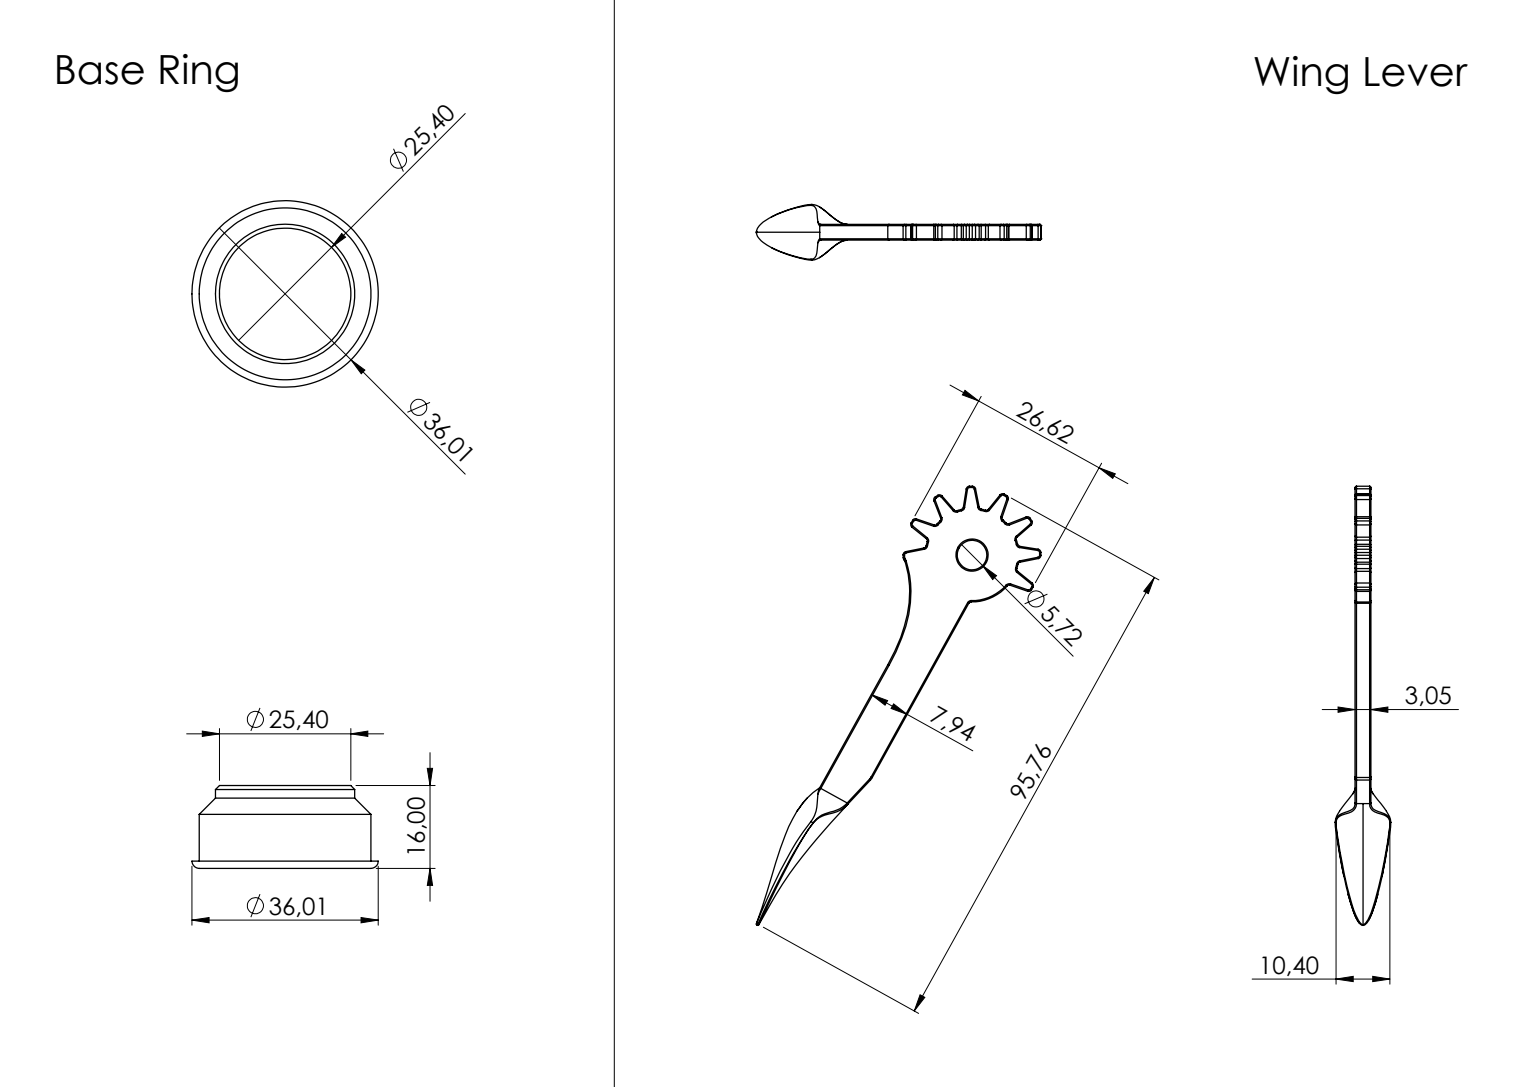
ISO-10303-21;
HEADER;
FILE_DESCRIPTION (('STEP AP214'),
    '1' );
FILE_NAME ('Base Ring.step',
    '2026-10-06T14:27:08',
    ( '' ),
    ( '' ),
    'SwSTEP 2.0',
    'SolidWorks 2020',
    '' );
FILE_SCHEMA (( 'AUTOMOTIVE_DESIGN' ));
ENDSEC;

DATA;
#28=SHAPE_DEFINITION_REPRESENTATION ( #10271, #23419 ) ;
#104=EDGE_LOOP ( 'NONE', ( #16225, #25822, #7892, #35896 ) ) ;
#162=DIRECTION ( 'NONE',  ( -1.000000000000000000, 1.365923996832131856E-16, 0.000000000000000000 ) ) ;
#198=EDGE_CURVE ( 'NONE', #31926, #33162, #2052, .T. ) ;
#286=EDGE_LOOP ( 'NONE', ( #24202, #14041, #34463, #28082 ) ) ;
#492=CONICAL_SURFACE ( 'NONE', #1854, 13.46199999999999619, 0.7853981633974482790 ) ;
#533=DIRECTION ( 'NONE',  ( -1.000000000000000000, 1.011795553208986377E-16, 0.000000000000000000 ) ) ;
#578=( GEOMETRIC_REPRESENTATION_CONTEXT ( 3 ) GLOBAL_UNCERTAINTY_ASSIGNED_CONTEXT ( ( #38497 ) ) GLOBAL_UNIT_ASSIGNED_CONTEXT ( ( #8767, #25159, #21514 ) ) REPRESENTATION_CONTEXT ( 'NONE', 'WORKASPACE' ) );
#588=VERTEX_POINT ( 'NONE', #40151 ) ;
#941=DIRECTION ( 'NONE',  ( -0.7071067811865480168, -0.7071067811865470176, 8.659560562354937789E-17 ) ) ;
#958=EDGE_LOOP ( 'NONE', ( #31328, #8348, #40597, #40431 ) ) ;
#1091=DIRECTION ( 'NONE',  ( 1.011795553208986377E-16, 1.000000000000000000, -0.000000000000000000 ) ) ;
#1122=FACE_OUTER_BOUND ( 'NONE', #9226, .T. ) ;
#1125=PRODUCT ( 'Base Ring', 'Base Ring', '', ( #16178 ) ) ;
#1185=CIRCLE ( 'NONE', #18138, 15.21260244842765452 ) ;
#1237=APPLICATION_CONTEXT ( 'automotive_design' ) ;
#1281=DIRECTION ( 'NONE',  ( 1.011795553208986377E-16, 1.000000000000000000, -0.000000000000000000 ) ) ;
#1340=CIRCLE ( 'NONE', #32609, 1.396999999999998909 ) ;
#1509=AXIS2_PLACEMENT_3D ( 'NONE', #17697, #33711, #23885 ) ;
#1551=CARTESIAN_POINT ( 'NONE',  ( -12.69999999999999574, 11.53894877578617262, 1.555301434917138235E-15 ) ) ;
#1689=DIRECTION ( 'NONE',  ( -1.000000000000000000, 1.011795553208986254E-16, 0.000000000000000000 ) ) ;
#1839=AXIS2_PLACEMENT_3D ( 'NONE', #27524, #17706, #30706 ) ;
#1854=AXIS2_PLACEMENT_3D ( 'NONE', #40634, #8669, #34449 ) ;
#1869=CARTESIAN_POINT ( 'NONE',  ( 18.00660244842765323, 1.647546923381499288E-15, 2.205172805198582110E-15 ) ) ;
#1931=COLOUR_RGB ( '', 0.31764706, 0.68627451, 0.89019608) ;
#2033=CARTESIAN_POINT ( 'NONE',  ( -13.46199999999999442, 13.84300000000000530, 0.000000000000000000 ) ) ;
#2052=LINE ( 'NONE', #35065, #8782 ) ;
#2100=DIRECTION ( 'NONE',  ( -1.011795553208986377E-16, -1.000000000000000000, 0.000000000000000000 ) ) ;
#2133=CIRCLE ( 'NONE', #17762, 18.00660244842765323 ) ;
#2169=AXIS2_PLACEMENT_3D ( 'NONE', #13076, #6484, #533 ) ;
#2601=SURFACE_STYLE_FILL_AREA ( #38160 ) ;
#2646=DIRECTION ( 'NONE',  ( -1.000000000000000000, 1.044409991968847425E-16, 0.000000000000000000 ) ) ;
#2678=ADVANCED_FACE ( 'NONE', ( #33479 ), #7528, .F. ) ;
#2788=DIRECTION ( 'NONE',  ( -0.000000000000000000, 0.000000000000000000, -1.000000000000000000 ) ) ;
#2922=CARTESIAN_POINT ( 'NONE',  ( 9.132817075745611705E-16, 9.026346327358515609, 0.000000000000000000 ) ) ;
#2930=DIRECTION ( 'NONE',  ( 1.011795553208986377E-16, 1.000000000000000000, -0.000000000000000000 ) ) ;
#2981=ORIENTED_EDGE ( 'NONE', *, *, #20181, .F. ) ;
#3129=DIRECTION ( 'NONE',  ( 1.011795553208986377E-16, 1.000000000000000000, -0.000000000000000000 ) ) ;
#3137=UNCERTAINTY_MEASURE_WITH_UNIT (LENGTH_MEASURE( 1.000000000000000082E-05 ), #37495, 'distance_accuracy_value', 'NONE');
#3220=CIRCLE ( 'NONE', #34506, 13.46199999999999619 ) ;
#3275=AXIS2_PLACEMENT_3D ( 'NONE', #6670, #19223, #39468 ) ;
#3342=AXIS2_PLACEMENT_3D ( 'NONE', #39599, #30984, #26590 ) ;
#3463=LINE ( 'NONE', #9627, #40991 ) ;
#3898=AXIS2_PLACEMENT_3D ( 'NONE', #7215, #36601, #20801 ) ;
#3930=CARTESIAN_POINT ( 'NONE',  ( -16.60960244842765476, 9.026346327358517385, 2.034089647357696543E-15 ) ) ;
#3948=DIRECTION ( 'NONE',  ( -1.000000000000000000, 0.000000000000000000, 0.000000000000000000 ) ) ;
#4240=EDGE_CURVE ( 'NONE', #23948, #24265, #1340, .T. ) ;
#4263=DIRECTION ( 'NONE',  ( 1.000000000000000000, 0.000000000000000000, 1.224646799147353454E-16 ) ) ;
#4371=LINE ( 'NONE', #23927, #16491 ) ;
#4500=CARTESIAN_POINT ( 'NONE',  ( 15.21260244842765985, 17.14499999999999957, 1.863006489516811765E-15 ) ) ;
#4541=ADVANCED_FACE ( 'NONE', ( #17843, #14644 ), #37662, .F. ) ;
#4704=EDGE_CURVE ( 'NONE', #10936, #33175, #39589, .T. ) ;
#4748=LINE ( 'NONE', #1551, #15031 ) ;
#5010=AXIS2_PLACEMENT_3D ( 'NONE', #7418, #7626, #14203 ) ;
#5096=DIRECTION ( 'NONE',  ( 1.011795553208986377E-16, 1.000000000000000000, -0.000000000000000000 ) ) ;
#5140=ORIENTED_EDGE ( 'NONE', *, *, #34929, .F. ) ;
#5196=DIRECTION ( 'NONE',  ( -1.000000000000000000, 1.288607544181256449E-16, 0.000000000000000000 ) ) ;
#5379=DIRECTION ( 'NONE',  ( -1.000000000000000000, 1.140319995778305956E-16, 0.000000000000000000 ) ) ;
#5443=CARTESIAN_POINT ( 'NONE',  ( 0.000000000000000000, 0.000000000000000000, 0.000000000000000000 ) ) ;
#5642=AXIS2_PLACEMENT_3D ( 'NONE', #33119, #13299, #3948 ) ;
#5724=DIRECTION ( 'NONE',  ( 1.011795553208986377E-16, 1.000000000000000000, -0.000000000000000000 ) ) ;
#5865=EDGE_CURVE ( 'NONE', #10936, #33761, #11552, .T. ) ;
#6152=ADVANCED_FACE ( 'NONE', ( #40324 ), #11323, .T. ) ;
#6171=FACE_OUTER_BOUND ( 'NONE', #34367, .T. ) ;
#6277=DIRECTION ( 'NONE',  ( 1.011795553208986377E-16, 1.000000000000000000, -0.000000000000000000 ) ) ;
#6301=FACE_OUTER_BOUND ( 'NONE', #41934, .T. ) ;
#6389=( NAMED_UNIT ( * ) SI_UNIT ( $, .STERADIAN. ) SOLID_ANGLE_UNIT ( ) );
#6484=DIRECTION ( 'NONE',  ( 1.011795553208986377E-16, 1.000000000000000000, -0.000000000000000000 ) ) ;
#6536=EDGE_CURVE ( 'NONE', #40785, #9160, #1185, .T. ) ;
#6586=VECTOR ( 'NONE', #9513, 1000.000000000000000 ) ;
#6670=CARTESIAN_POINT ( 'NONE',  ( 0.000000000000000000, 0.000000000000000000, 0.000000000000000000 ) ) ;
#6769=CARTESIAN_POINT ( 'NONE',  ( -16.60960244842765121, 9.026346327358517385, 0.000000000000000000 ) ) ;
#6888=ORIENTED_EDGE ( 'NONE', *, *, #6536, .F. ) ;
#6966=UNCERTAINTY_MEASURE_WITH_UNIT (LENGTH_MEASURE( 1.000000000000000082E-05 ), #37731, 'distance_accuracy_value', 'NONE');
#7111=DIRECTION ( 'NONE',  ( 1.011795553208986377E-16, 1.000000000000000000, -0.000000000000000000 ) ) ;
#7121=EDGE_CURVE ( 'NONE', #33175, #10936, #23398, .T. ) ;
#7215=CARTESIAN_POINT ( 'NONE',  ( 0.000000000000000000, -2.099656937138137170E-16, 0.000000000000000000 ) ) ;
#7291=VECTOR ( 'NONE', #19971, 999.9999999999998863 ) ;
#7323=VECTOR ( 'NONE', #17892, 1000.000000000000000 ) ;
#7418=CARTESIAN_POINT ( 'NONE',  ( 1.400628584307200167E-15, 13.84300000000000352, 0.000000000000000000 ) ) ;
#7528=CONICAL_SURFACE ( 'NONE', #27261, 12.69999999999999751, 0.7853981633974485010 ) ;
#7537=DIRECTION ( 'NONE',  ( -0.7071067811865475727, -0.7071067811865474617, 8.659560562354931626E-17 ) ) ;
#7626=DIRECTION ( 'NONE',  ( 1.011795553208986377E-16, 1.000000000000000000, -0.000000000000000000 ) ) ;
#7692=ADVANCED_FACE ( 'NONE', ( #30190 ), #15882, .T. ) ;
#7734=CIRCLE ( 'NONE', #5010, 13.46199999999999619 ) ;
#7767=CIRCLE ( 'NONE', #34285, 16.60960244842765121 ) ;
#7855=ORIENTED_EDGE ( 'NONE', *, *, #29567, .F. ) ;
#7892=ORIENTED_EDGE ( 'NONE', *, *, #14938, .T. ) ;
#7966=ORIENTED_EDGE ( 'NONE', *, *, #39208, .F. ) ;
#8152=CIRCLE ( 'NONE', #41493, 12.69999999999999751 ) ;
#8348=ORIENTED_EDGE ( 'NONE', *, *, #10985, .F. ) ;
#8436=DIRECTION ( 'NONE',  ( 0.7071067811865479058, -0.7071067811865472397, 0.000000000000000000 ) ) ;
#8650=ORIENTED_EDGE ( 'NONE', *, *, #10267, .F. ) ;
#8669=DIRECTION ( 'NONE',  ( -1.011795553208986377E-16, -1.000000000000000000, 0.000000000000000000 ) ) ;
#8741=LINE ( 'NONE', #27698, #7323 ) ;
#8767=( LENGTH_UNIT ( ) NAMED_UNIT ( * ) SI_UNIT ( .MILLI., .METRE. ) );
#8782=VECTOR ( 'NONE', #8436, 999.9999999999998863 ) ;
#9017=ORIENTED_EDGE ( 'NONE', *, *, #20410, .F. ) ;
#9030=CARTESIAN_POINT ( 'NONE',  ( 1.925929944387235853E-31, 3.469446951953614189E-15, 0.000000000000000000 ) ) ;
#9144=VERTEX_POINT ( 'NONE', #33041 ) ;
#9160=VERTEX_POINT ( 'NONE', #26423 ) ;
#9167=PRESENTATION_STYLE_ASSIGNMENT (( #18942 ) ) ;
#9226=EDGE_LOOP ( 'NONE', ( #39033, #15868, #33796, #5140 ) ) ;
#9235=DIRECTION ( 'NONE',  ( 1.011795553208986377E-16, 1.000000000000000000, -0.000000000000000000 ) ) ;
#9399=( GEOMETRIC_REPRESENTATION_CONTEXT ( 3 ) GLOBAL_UNCERTAINTY_ASSIGNED_CONTEXT ( ( #6966 ) ) GLOBAL_UNIT_ASSIGNED_CONTEXT ( ( #37731, #25368, #30916 ) ) REPRESENTATION_CONTEXT ( 'NONE', 'WORKASPACE' ) );
#9512=LINE ( 'NONE', #22900, #23306 ) ;
#9513=DIRECTION ( 'NONE',  ( 1.011795553208986377E-16, 1.000000000000000000, -0.000000000000000000 ) ) ;
#9578=DIRECTION ( 'NONE',  ( 1.011795553208986377E-16, 1.000000000000000000, -0.000000000000000000 ) ) ;
#9627=CARTESIAN_POINT ( 'NONE',  ( 12.69999999999999929, 11.53894877578616907, 0.000000000000000000 ) ) ;
#9924=FACE_OUTER_BOUND ( 'NONE', #958, .T. ) ;
#10000=CARTESIAN_POINT ( 'NONE',  ( 13.46199999999999797, 12.17394877578616885, 0.000000000000000000 ) ) ;
#10042=EDGE_CURVE ( 'NONE', #23250, #33175, #29354, .T. ) ;
#10074=CARTESIAN_POINT ( 'NONE',  ( 1.734723475976807094E-15, 17.14499999999999957, 0.000000000000000000 ) ) ;
#10090=ADVANCED_FACE ( 'NONE', ( #14413 ), #35845, .T. ) ;
#10267=EDGE_CURVE ( 'NONE', #33175, #38422, #27212, .T. ) ;
#10271=PRODUCT_DEFINITION_SHAPE ( 'NONE', 'NONE',  #24009 ) ;
#10279=EDGE_LOOP ( 'NONE', ( #25889, #32003, #13465, #38023 ) ) ;
#10314=CYLINDRICAL_SURFACE ( 'NONE', #5642, 12.69999999999999751 ) ;
#10358=CIRCLE ( 'NONE', #20532, 13.46199999999999619 ) ;
#10433=ORIENTED_EDGE ( 'NONE', *, *, #36513, .F. ) ;
#10440=DIRECTION ( 'NONE',  ( -1.000000000000000000, 1.365923996832131856E-16, 0.000000000000000000 ) ) ;
#10450=AXIS2_PLACEMENT_3D ( 'NONE', #23996, #40222, #33612 ) ;
#10549=ADVANCED_FACE ( 'NONE', ( #24418 ), #492, .T. ) ;
#10595=CARTESIAN_POINT ( 'NONE',  ( 1.734723475976807094E-15, 17.14499999999999957, 0.000000000000000000 ) ) ;
#10680=AXIS2_PLACEMENT_3D ( 'NONE', #2922, #35291, #38487 ) ;
#10710=DIRECTION ( 'NONE',  ( 1.011795553208986377E-16, 1.000000000000000000, -0.000000000000000000 ) ) ;
#10741=ORIENTED_EDGE ( 'NONE', *, *, #29867, .F. ) ;
#10841=CYLINDRICAL_SURFACE ( 'NONE', #19739, 13.46199999999999619 ) ;
#10929=DIRECTION ( 'NONE',  ( 1.011795553208986377E-16, 1.000000000000000000, -0.000000000000000000 ) ) ;
#10936=VERTEX_POINT ( 'NONE', #12703 ) ;
#10967=ADVANCED_FACE ( 'NONE', ( #9924 ), #13428, .T. ) ;
#10985=EDGE_CURVE ( 'NONE', #31926, #588, #3220, .T. ) ;
#11014=ORIENTED_EDGE ( 'NONE', *, *, #198, .F. ) ;
#11115=STYLED_ITEM ( 'NONE', ( #9167 ), #24724 ) ;
#11209=ORIENTED_EDGE ( 'NONE', *, *, #4240, .F. ) ;
#11323=CYLINDRICAL_SURFACE ( 'NONE', #1839, 16.60960244842765832 ) ;
#11522=DIRECTION ( 'NONE',  ( 1.000000000000000000, -1.288607544181256449E-16, 0.000000000000000000 ) ) ;
#11552=LINE ( 'NONE', #24535, #32246 ) ;
#11622=CARTESIAN_POINT ( 'NONE',  ( 12.69999999999999929, 11.53894877578616907, 1.555301434917138235E-15 ) ) ;
#11697=ORIENTED_EDGE ( 'NONE', *, *, #27784, .F. ) ;
#11747=DIRECTION ( 'NONE',  ( 1.011795553208986377E-16, 1.000000000000000000, -0.000000000000000000 ) ) ;
#11922=ORIENTED_EDGE ( 'NONE', *, *, #38918, .T. ) ;
#11949=ORIENTED_EDGE ( 'NONE', *, *, #30623, .F. ) ;
#12198=CARTESIAN_POINT ( 'NONE',  ( 13.46199999999999797, 17.14499999999999957, 1.648619521012166368E-15 ) ) ;
#12391=ORIENTED_EDGE ( 'NONE', *, *, #5865, .T. ) ;
#12509=ORIENTED_EDGE ( 'NONE', *, *, #7121, .F. ) ;
#12518=CARTESIAN_POINT ( 'NONE',  ( 15.21260244842765808, -1.539204351005524363E-15, 1.863006489516811765E-15 ) ) ;
#12579=ORIENTED_EDGE ( 'NONE', *, *, #39208, .T. ) ;
#12703=CARTESIAN_POINT ( 'NONE',  ( -12.69999999999999574, 14.60500000000000398, 1.601960477964652499E-15 ) ) ;
#12711=CARTESIAN_POINT ( 'NONE',  ( 1.167505706004672243E-15, 11.53894877578617084, 0.000000000000000000 ) ) ;
#12917=PRODUCT_DEFINITION_CONTEXT ( 'detailed design', #1237, 'design' ) ;
#12967=VECTOR ( 'NONE', #1091, 1000.000000000000000 ) ;
#12972=DIRECTION ( 'NONE',  ( -1.000000000000000000, 0.000000000000000000, 0.000000000000000000 ) ) ;
#13028=EDGE_CURVE ( 'NONE', #33162, #41686, #7767, .T. ) ;
#13076=CARTESIAN_POINT ( 'NONE',  ( 0.000000000000000000, 0.000000000000000000, 0.000000000000000000 ) ) ;
#13133=CONICAL_SURFACE ( 'NONE', #38322, 16.60960244842765476, 0.7853981633974488341 ) ;
#13166=ORIENTED_EDGE ( 'NONE', *, *, #7121, .T. ) ;
#13299=DIRECTION ( 'NONE',  ( 1.011795553208986377E-16, 1.000000000000000000, -0.000000000000000000 ) ) ;
#13342=CARTESIAN_POINT ( 'NONE',  ( -13.46199999999999442, 17.14499999999999957, 0.000000000000000000 ) ) ;
#13405=DIRECTION ( 'NONE',  ( -1.000000000000000000, 1.011795553208986377E-16, 0.000000000000000000 ) ) ;
#13428=CONICAL_SURFACE ( 'NONE', #10680, 16.60960244842765476, 0.7853981633974488341 ) ;
#13465=ORIENTED_EDGE ( 'NONE', *, *, #20356, .T. ) ;
#13483=MECHANICAL_DESIGN_GEOMETRIC_PRESENTATION_REPRESENTATION('',(#26389),#578);
#13490=CYLINDRICAL_SURFACE ( 'NONE', #34725, 12.69999999999999751 ) ;
#13722=EDGE_LOOP ( 'NONE', ( #11697, #24432, #41846, #6888 ) ) ;
#13911=CARTESIAN_POINT ( 'NONE',  ( 1.734723475976807094E-15, 17.14499999999999957, 0.000000000000000000 ) ) ;
#14027=CARTESIAN_POINT ( 'NONE',  ( 16.60960244842765832, -1.890517883502633324E-15, 2.034089647357696937E-15 ) ) ;
#14041=ORIENTED_EDGE ( 'NONE', *, *, #34939, .F. ) ;
#14060=AXIS2_PLACEMENT_3D ( 'NONE', #30575, #17370, #17160 ) ;
#14092=CARTESIAN_POINT ( 'NONE',  ( 16.60960244842765121, 9.026346327358513832, 2.034089647357696543E-15 ) ) ;
#14189=EDGE_LOOP ( 'NONE', ( #11922, #16644, #17909, #26794 ) ) ;
#14199=AXIS2_PLACEMENT_3D ( 'NONE', #16142, #25740, #29144 ) ;
#14203=DIRECTION ( 'NONE',  ( -1.000000000000000000, 1.288607544181256449E-16, 0.000000000000000000 ) ) ;
#14257=EDGE_LOOP ( 'NONE', ( #20749, #12579, #31415, #11209 ) ) ;
#14298=AXIS2_PLACEMENT_3D ( 'NONE', #24726, #33916, #11522 ) ;
#14315=ADVANCED_FACE ( 'NONE', ( #33834 ), #13133, .T. ) ;
#14395=ORIENTED_EDGE ( 'NONE', *, *, #18291, .T. ) ;
#14413=FACE_OUTER_BOUND ( 'NONE', #14257, .T. ) ;
#14500=ORIENTED_EDGE ( 'NONE', *, *, #4704, .F. ) ;
#14644=FACE_OUTER_BOUND ( 'NONE', #14920, .T. ) ;
#14895=EDGE_LOOP ( 'NONE', ( #14500, #12391, #22139, #8650 ) ) ;
#14920=EDGE_LOOP ( 'NONE', ( #41142, #40216 ) ) ;
#14938=EDGE_CURVE ( 'NONE', #23948, #40785, #9512, .T. ) ;
#15031=VECTOR ( 'NONE', #31333, 999.9999999999998863 ) ;
#15134=SURFACE_STYLE_USAGE ( .BOTH. , #18750 ) ;
#15308=ADVANCED_BREP_SHAPE_REPRESENTATION ( '', ( #24724, #3275 ), #9399 ) ;
#15318=ORIENTED_EDGE ( 'NONE', *, *, #10042, .T. ) ;
#15348=SHAPE_REPRESENTATION_RELATIONSHIP ( 'NONE' , 'NONE' ,  #23419, #15308 ) ;
#15450=DIRECTION ( 'NONE',  ( -1.000000000000000000, 1.365923996832131856E-16, 0.000000000000000000 ) ) ;
#15609=DIRECTION ( 'NONE',  ( -1.000000000000000000, 1.011795553208986377E-16, 0.000000000000000000 ) ) ;
#15868=ORIENTED_EDGE ( 'NONE', *, *, #29567, .T. ) ;
#15882=TOROIDAL_SURFACE ( 'NONE', #10450, 16.60960244842765832, 1.396999999999998909 ) ;
#15957=DIRECTION ( 'NONE',  ( -1.000000000000000000, 1.011795553208986254E-16, 0.000000000000000000 ) ) ;
#15991=EDGE_CURVE ( 'NONE', #33761, #38422, #7734, .T. ) ;
#16012=ORIENTED_EDGE ( 'NONE', *, *, #35198, .T. ) ;
#16134=ADVANCED_FACE ( 'NONE', ( #30397 ), #24206, .F. ) ;
#16142=CARTESIAN_POINT ( 'NONE',  ( 1.734723475976807094E-15, 17.14499999999999957, 0.000000000000000000 ) ) ;
#16160=CARTESIAN_POINT ( 'NONE',  ( 0.000000000000000000, 0.000000000000000000, 0.000000000000000000 ) ) ;
#16178=PRODUCT_CONTEXT ( 'NONE', #35495, 'mechanical' ) ;
#16225=ORIENTED_EDGE ( 'NONE', *, *, #18291, .F. ) ;
#16283=DIRECTION ( 'NONE',  ( 1.000000000000000000, -1.365923996832131856E-16, 0.000000000000000000 ) ) ;
#16491=VECTOR ( 'NONE', #24549, 1000.000000000000000 ) ;
#16565=DIRECTION ( 'NONE',  ( 1.011795553208986377E-16, 1.000000000000000000, -0.000000000000000000 ) ) ;
#16644=ORIENTED_EDGE ( 'NONE', *, *, #31107, .T. ) ;
#16881=EDGE_LOOP ( 'NONE', ( #7966, #38209, #30590, #22905 ) ) ;
#17160=DIRECTION ( 'NONE',  ( -1.000000000000000000, 1.044409991968847425E-16, 0.000000000000000000 ) ) ;
#17274=DIRECTION ( 'NONE',  ( 1.000000000000000000, -1.365923996832131856E-16, 0.000000000000000000 ) ) ;
#17370=DIRECTION ( 'NONE',  ( 1.011795553208986377E-16, 1.000000000000000000, -0.000000000000000000 ) ) ;
#17495=CYLINDRICAL_SURFACE ( 'NONE', #1509, 13.46199999999999619 ) ;
#17510=ADVANCED_FACE ( 'NONE', ( #39268 ), #13490, .F. ) ;
#17697=CARTESIAN_POINT ( 'NONE',  ( 1.734723475976807094E-15, 17.14499999999999957, 0.000000000000000000 ) ) ;
#17706=DIRECTION ( 'NONE',  ( 1.011795553208986377E-16, 1.000000000000000000, -0.000000000000000000 ) ) ;
#17762=AXIS2_PLACEMENT_3D ( 'NONE', #9030, #21995, #15609 ) ;
#17829=DIRECTION ( 'NONE',  ( -1.011795553208986377E-16, -1.000000000000000000, 0.000000000000000000 ) ) ;
#17843=FACE_BOUND ( 'NONE', #31275, .T. ) ;
#17892=DIRECTION ( 'NONE',  ( 1.011795553208986377E-16, 1.000000000000000000, -0.000000000000000000 ) ) ;
#17909=ORIENTED_EDGE ( 'NONE', *, *, #35198, .F. ) ;
#18138=AXIS2_PLACEMENT_3D ( 'NONE', #34977, #11747, #5379 ) ;
#18291=EDGE_CURVE ( 'NONE', #22322, #9160, #32610, .T. ) ;
#18359=DIRECTION ( 'NONE',  ( 1.011795553208986377E-16, 1.000000000000000000, -0.000000000000000000 ) ) ;
#18467=ORIENTED_EDGE ( 'NONE', *, *, #10267, .T. ) ;
#18517=FILL_AREA_STYLE ('',( #41124 ) ) ;
#18750=SURFACE_SIDE_STYLE ('',( #2601 ) ) ;
#18935=CIRCLE ( 'NONE', #33930, 15.21260244842765808 ) ;
#18942=SURFACE_STYLE_USAGE ( .BOTH. , #38350 ) ;
#19078=CONICAL_SURFACE ( 'NONE', #14298, 13.46199999999999619, 0.7853981633974482790 ) ;
#19223=DIRECTION ( 'NONE',  ( 0.000000000000000000, 0.000000000000000000, 1.000000000000000000 ) ) ;
#19360=CARTESIAN_POINT ( 'NONE',  ( -16.60960244842765832, 1.470586496075005742E-15, 0.000000000000000000 ) ) ;
#19534=VERTEX_POINT ( 'NONE', #1869 ) ;
#19624=CARTESIAN_POINT ( 'NONE',  ( 16.60960244842765832, -1.680552189788819435E-15, 2.034089647357696937E-15 ) ) ;
#19739=AXIS2_PLACEMENT_3D ( 'NONE', #23826, #1281, #24040 ) ;
#19971=DIRECTION ( 'NONE',  ( 0.7071067811865473507, -0.7071067811865477948, 0.000000000000000000 ) ) ;
#20069=DIRECTION ( 'NONE',  ( -1.000000000000000000, 0.000000000000000000, 0.000000000000000000 ) ) ;
#20077=DIRECTION ( 'NONE',  ( -1.000000000000000000, 0.000000000000000000, 0.000000000000000000 ) ) ;
#20132=ADVANCED_FACE ( 'NONE', ( #6171 ), #22528, .F. ) ;
#20181=EDGE_CURVE ( 'NONE', #38422, #33761, #27130, .T. ) ;
#20211=CONICAL_SURFACE ( 'NONE', #22239, 12.69999999999999751, 0.7853981633974485010 ) ;
#20356=EDGE_CURVE ( 'NONE', #9144, #41686, #34615, .T. ) ;
#20376=DIRECTION ( 'NONE',  ( 1.011795553208986377E-16, 1.000000000000000000, -0.000000000000000000 ) ) ;
#20410=EDGE_CURVE ( 'NONE', #22322, #23948, #18935, .T. ) ;
#20503=CARTESIAN_POINT ( 'NONE',  ( 1.231754723633442730E-15, 12.17394877578617063, 0.000000000000000000 ) ) ;
#20532=AXIS2_PLACEMENT_3D ( 'NONE', #20503, #10929, #5196 ) ;
#20585=DIRECTION ( 'NONE',  ( -1.000000000000000000, 0.000000000000000000, 0.000000000000000000 ) ) ;
#20749=ORIENTED_EDGE ( 'NONE', *, *, #28749, .T. ) ;
#20767=AXIS2_PLACEMENT_3D ( 'NONE', #14027, #37049, #4263 ) ;
#20801=DIRECTION ( 'NONE',  ( -1.000000000000000000, 1.011795553208986254E-16, 0.000000000000000000 ) ) ;
#20952=VECTOR ( 'NONE', #16565, 1000.000000000000000 ) ;
#21022=CARTESIAN_POINT ( 'NONE',  ( 13.46199999999999797, 13.84300000000000175, 1.648619521012166368E-15 ) ) ;
#21239=DIRECTION ( 'NONE',  ( 1.000000000000000000, -1.011795553208986377E-16, 0.000000000000000000 ) ) ;
#21514=( NAMED_UNIT ( * ) SI_UNIT ( $, .STERADIAN. ) SOLID_ANGLE_UNIT ( ) );
#21727=PRESENTATION_STYLE_ASSIGNMENT (( #15134 ) ) ;
#21995=DIRECTION ( 'NONE',  ( 1.011795553208986377E-16, 1.000000000000000000, -0.000000000000000000 ) ) ;
#22133=EDGE_LOOP ( 'NONE', ( #38843, #12509, #18467, #34287 ) ) ;
#22139=ORIENTED_EDGE ( 'NONE', *, *, #15991, .T. ) ;
#22194=CIRCLE ( 'NONE', #30393, 12.69999999999999751 ) ;
#22239=AXIS2_PLACEMENT_3D ( 'NONE', #28451, #29073, #16283 ) ;
#22322=VERTEX_POINT ( 'NONE', #12518 ) ;
#22528=CYLINDRICAL_SURFACE ( 'NONE', #14199, 15.21260244842765808 ) ;
#22594=DIRECTION ( 'NONE',  ( 0.7071067811865475727, -0.7071067811865474617, 0.000000000000000000 ) ) ;
#22608=EDGE_LOOP ( 'NONE', ( #35370, #35414, #16012, #11014 ) ) ;
#22740=ORIENTED_EDGE ( 'NONE', *, *, #24798, .F. ) ;
#22792=CIRCLE ( 'NONE', #20767, 1.396999999999998909 ) ;
#22900=CARTESIAN_POINT ( 'NONE',  ( -15.21260244842765630, 17.14499999999999957, 0.000000000000000000 ) ) ;
#22905=ORIENTED_EDGE ( 'NONE', *, *, #38951, .F. ) ;
#22938=CARTESIAN_POINT ( 'NONE',  ( 12.69999999999999929, 17.14499999999999957, 1.555301434917138235E-15 ) ) ;
#22965=CARTESIAN_POINT ( 'NONE',  ( 1.925929944387235853E-31, 3.469446951953614189E-15, 0.000000000000000000 ) ) ;
#23212=EDGE_CURVE ( 'NONE', #23250, #28134, #8152, .T. ) ;
#23219=AXIS2_PLACEMENT_3D ( 'NONE', #24233, #2100, #21239 ) ;
#23250=VERTEX_POINT ( 'NONE', #11622 ) ;
#23306=VECTOR ( 'NONE', #32518, 1000.000000000000000 ) ;
#23398=CIRCLE ( 'NONE', #29538, 12.69999999999999751 ) ;
#23419=SHAPE_REPRESENTATION ( 'Base Ring', ( #3275 ), #9399 ) ;
#23758=DIRECTION ( 'NONE',  ( 1.011795553208986377E-16, 1.000000000000000000, -0.000000000000000000 ) ) ;
#23826=CARTESIAN_POINT ( 'NONE',  ( 1.734723475976807094E-15, 17.14499999999999957, 0.000000000000000000 ) ) ;
#23885=DIRECTION ( 'NONE',  ( -1.000000000000000000, 0.000000000000000000, 0.000000000000000000 ) ) ;
#23927=CARTESIAN_POINT ( 'NONE',  ( 16.60960244842765832, 17.14499999999999957, 2.034089647357696937E-15 ) ) ;
#23948=VERTEX_POINT ( 'NONE', #25795 ) ;
#23971=ORIENTED_EDGE ( 'NONE', *, *, #38918, .F. ) ;
#23996=CARTESIAN_POINT ( 'NONE',  ( 0.000000000000000000, -2.099656937138137170E-16, 0.000000000000000000 ) ) ;
#24009=PRODUCT_DEFINITION ( 'UNKNOWN', '', #40070, #12917 ) ;
#24040=DIRECTION ( 'NONE',  ( -1.000000000000000000, 0.000000000000000000, 0.000000000000000000 ) ) ;
#24202=ORIENTED_EDGE ( 'NONE', *, *, #10042, .F. ) ;
#24206=CYLINDRICAL_SURFACE ( 'NONE', #30821, 15.21260244842765808 ) ;
#24233=CARTESIAN_POINT ( 'NONE',  ( 16.60960244842765832, -1.392917743221662552E-16, 0.000000000000000000 ) ) ;
#24265=VERTEX_POINT ( 'NONE', #31731 ) ;
#24418=FACE_OUTER_BOUND ( 'NONE', #22133, .T. ) ;
#24432=ORIENTED_EDGE ( 'NONE', *, *, #34939, .T. ) ;
#24441=CARTESIAN_POINT ( 'NONE',  ( 1.477727405461724555E-15, 14.60500000000000220, 0.000000000000000000 ) ) ;
#24535=CARTESIAN_POINT ( 'NONE',  ( -13.46199999999999442, 13.84300000000000530, 1.648619521012166368E-15 ) ) ;
#24549=DIRECTION ( 'NONE',  ( 1.011795553208986377E-16, 1.000000000000000000, -0.000000000000000000 ) ) ;
#24724=MANIFOLD_SOLID_BREP ( 'Stock-MAS-162-1', #27830 ) ;
#24726=CARTESIAN_POINT ( 'NONE',  ( 1.400628584307200167E-15, 13.84300000000000352, 0.000000000000000000 ) ) ;
#24728=FILL_AREA_STYLE_COLOUR ( '', #1931 ) ;
#24798=EDGE_CURVE ( 'NONE', #31688, #9144, #39006, .T. ) ;
#24826=CARTESIAN_POINT ( 'NONE',  ( 1.167505706004672243E-15, 11.53894877578617084, 0.000000000000000000 ) ) ;
#24953=AXIS2_PLACEMENT_3D ( 'NONE', #13911, #10710, #20077 ) ;
#25015=DIRECTION ( 'NONE',  ( -1.000000000000000000, 1.011795553208986377E-16, 0.000000000000000000 ) ) ;
#25159=( NAMED_UNIT ( * ) PLANE_ANGLE_UNIT ( ) SI_UNIT ( $, .RADIAN. ) );
#25161=CARTESIAN_POINT ( 'NONE',  ( -12.69999999999999574, 11.53894877578617262, 0.000000000000000000 ) ) ;
#25255=ORIENTED_EDGE ( 'NONE', *, *, #23212, .T. ) ;
#25368=( NAMED_UNIT ( * ) PLANE_ANGLE_UNIT ( ) SI_UNIT ( $, .RADIAN. ) );
#25383=MECHANICAL_DESIGN_GEOMETRIC_PRESENTATION_REPRESENTATION('',(#11115),#38309);
#25406=LINE ( 'NONE', #12198, #31425 ) ;
#25528=ORIENTED_EDGE ( 'NONE', *, *, #30623, .T. ) ;
#25740=DIRECTION ( 'NONE',  ( 1.011795553208986377E-16, 1.000000000000000000, -0.000000000000000000 ) ) ;
#25795=CARTESIAN_POINT ( 'NONE',  ( -15.21260244842765808, 1.539204351005524363E-15, 0.000000000000000000 ) ) ;
#25822=ORIENTED_EDGE ( 'NONE', *, *, #28749, .F. ) ;
#25889=ORIENTED_EDGE ( 'NONE', *, *, #31107, .F. ) ;
#26178=CARTESIAN_POINT ( 'NONE',  ( 9.132817075745611705E-16, 9.026346327358515609, 0.000000000000000000 ) ) ;
#26329=LINE ( 'NONE', #13342, #6586 ) ;
#26389=STYLED_ITEM ( 'NONE', ( #21727 ), #15308 ) ;
#26423=CARTESIAN_POINT ( 'NONE',  ( 15.21260244842765452, 9.026346327358513832, 0.000000000000000000 ) ) ;
#26590=DIRECTION ( 'NONE',  ( -1.000000000000000000, 1.288607544181256449E-16, 0.000000000000000000 ) ) ;
#26650=DIRECTION ( 'NONE',  ( -1.011795553208986377E-16, -1.000000000000000000, 0.000000000000000000 ) ) ;
#26794=ORIENTED_EDGE ( 'NONE', *, *, #20356, .F. ) ;
#26897=CIRCLE ( 'NONE', #32336, 16.60960244842765832 ) ;
#27130=CIRCLE ( 'NONE', #3342, 13.46199999999999619 ) ;
#27212=LINE ( 'NONE', #40227, #7291 ) ;
#27261=AXIS2_PLACEMENT_3D ( 'NONE', #36461, #26650, #17274 ) ;
#27302=FACE_OUTER_BOUND ( 'NONE', #14895, .T. ) ;
#27436=EDGE_CURVE ( 'NONE', #24265, #19534, #2133, .T. ) ;
#27473=DIRECTION ( 'NONE',  ( 1.011795553208986377E-16, 1.000000000000000000, -0.000000000000000000 ) ) ;
#27524=CARTESIAN_POINT ( 'NONE',  ( 1.734723475976807094E-15, 17.14499999999999957, 0.000000000000000000 ) ) ;
#27570=AXIS2_PLACEMENT_3D ( 'NONE', #22965, #35576, #13405 ) ;
#27698=CARTESIAN_POINT ( 'NONE',  ( -12.69999999999999574, 17.14499999999999957, 0.000000000000000000 ) ) ;
#27784=EDGE_CURVE ( 'NONE', #28134, #40785, #4748, .T. ) ;
#27830=CLOSED_SHELL ( 'NONE', ( #10090, #20132, #40282, #17510, #33005, #32951, #14315, #34517, #4541, #6152, #10967, #32221, #10549, #31035, #2678, #16134, #7692 ) ) ;
#28082=ORIENTED_EDGE ( 'NONE', *, *, #4704, .T. ) ;
#28134=VERTEX_POINT ( 'NONE', #25161 ) ;
#28323=CIRCLE ( 'NONE', #14060, 16.60960244842765121 ) ;
#28349=EDGE_LOOP ( 'NONE', ( #7855, #41999, #38886, #2981 ) ) ;
#28451=CARTESIAN_POINT ( 'NONE',  ( 1.167505706004672243E-15, 11.53894877578617084, 0.000000000000000000 ) ) ;
#28749=EDGE_CURVE ( 'NONE', #23948, #22322, #29357, .T. ) ;
#29029=EDGE_LOOP ( 'NONE', ( #39414, #15318, #13166, #10433 ) ) ;
#29073=DIRECTION ( 'NONE',  ( -1.011795553208986377E-16, -1.000000000000000000, 0.000000000000000000 ) ) ;
#29144=DIRECTION ( 'NONE',  ( -1.000000000000000000, 0.000000000000000000, 0.000000000000000000 ) ) ;
#29256=EDGE_CURVE ( 'NONE', #588, #31926, #10358, .T. ) ;
#29354=LINE ( 'NONE', #22938, #20952 ) ;
#29357=CIRCLE ( 'NONE', #2169, 15.21260244842765808 ) ;
#29503=CARTESIAN_POINT ( 'NONE',  ( -15.21260244842765275, 9.026346327358517385, 1.863006489516811765E-15 ) ) ;
#29538=AXIS2_PLACEMENT_3D ( 'NONE', #36442, #27473, #10440 ) ;
#29567=EDGE_CURVE ( 'NONE', #31926, #38422, #25406, .T. ) ;
#29867=EDGE_CURVE ( 'NONE', #23250, #9160, #3463, .T. ) ;
#30101=CYLINDRICAL_SURFACE ( 'NONE', #24953, 16.60960244842765832 ) ;
#30167=DIRECTION ( 'NONE',  ( -1.000000000000000000, 1.140319995778305956E-16, 0.000000000000000000 ) ) ;
#30190=FACE_OUTER_BOUND ( 'NONE', #16881, .T. ) ;
#30393=AXIS2_PLACEMENT_3D ( 'NONE', #12711, #2930, #162 ) ;
#30397=FACE_OUTER_BOUND ( 'NONE', #104, .T. ) ;
#30575=CARTESIAN_POINT ( 'NONE',  ( 9.132817075745611705E-16, 9.026346327358515609, 0.000000000000000000 ) ) ;
#30590=ORIENTED_EDGE ( 'NONE', *, *, #4240, .T. ) ;
#30623=EDGE_CURVE ( 'NONE', #9160, #40785, #36916, .T. ) ;
#30706=DIRECTION ( 'NONE',  ( -1.000000000000000000, 0.000000000000000000, 0.000000000000000000 ) ) ;
#30821=AXIS2_PLACEMENT_3D ( 'NONE', #10595, #20376, #20585 ) ;
#30916=( NAMED_UNIT ( * ) SI_UNIT ( $, .STERADIAN. ) SOLID_ANGLE_UNIT ( ) );
#30984=DIRECTION ( 'NONE',  ( 1.011795553208986377E-16, 1.000000000000000000, -0.000000000000000000 ) ) ;
#31035=ADVANCED_FACE ( 'NONE', ( #32906 ), #10314, .F. ) ;
#31107=EDGE_CURVE ( 'NONE', #31688, #33162, #4371, .T. ) ;
#31275=EDGE_LOOP ( 'NONE', ( #23971, #22740 ) ) ;
#31328=ORIENTED_EDGE ( 'NONE', *, *, #34455, .F. ) ;
#31333=DIRECTION ( 'NONE',  ( -0.7071067811865479058, -0.7071067811865472397, 8.659560562354936556E-17 ) ) ;
#31415=ORIENTED_EDGE ( 'NONE', *, *, #27436, .F. ) ;
#31425=VECTOR ( 'NONE', #18359, 1000.000000000000000 ) ;
#31647=DIRECTION ( 'NONE',  ( 1.011795553208986377E-16, 1.000000000000000000, -0.000000000000000000 ) ) ;
#31688=VERTEX_POINT ( 'NONE', #19624 ) ;
#31731=CARTESIAN_POINT ( 'NONE',  ( -18.00660244842765323, 5.291346980525729287E-15, 0.000000000000000000 ) ) ;
#31926=VERTEX_POINT ( 'NONE', #10000 ) ;
#32003=ORIENTED_EDGE ( 'NONE', *, *, #24798, .T. ) ;
#32221=ADVANCED_FACE ( 'NONE', ( #33233 ), #10841, .T. ) ;
#32246=VECTOR ( 'NONE', #7537, 1000.000000000000000 ) ;
#32299=CARTESIAN_POINT ( 'NONE',  ( 1.231754723633442730E-15, 12.17394877578617063, 0.000000000000000000 ) ) ;
#32336=AXIS2_PLACEMENT_3D ( 'NONE', #16160, #9578, #15957 ) ;
#32518=DIRECTION ( 'NONE',  ( 1.011795553208986377E-16, 1.000000000000000000, -0.000000000000000000 ) ) ;
#32563=ORIENTED_EDGE ( 'NONE', *, *, #27784, .T. ) ;
#32609=AXIS2_PLACEMENT_3D ( 'NONE', #19360, #2788, #12972 ) ;
#32610=LINE ( 'NONE', #4500, #12967 ) ;
#32906=FACE_OUTER_BOUND ( 'NONE', #286, .T. ) ;
#32951=ADVANCED_FACE ( 'NONE', ( #1122 ), #17495, .T. ) ;
#33005=ADVANCED_FACE ( 'NONE', ( #27302 ), #19078, .T. ) ;
#33041=CARTESIAN_POINT ( 'NONE',  ( -16.60960244842765832, 1.680552189788819435E-15, 0.000000000000000000 ) ) ;
#33119=CARTESIAN_POINT ( 'NONE',  ( 1.734723475976807094E-15, 17.14499999999999957, 0.000000000000000000 ) ) ;
#33162=VERTEX_POINT ( 'NONE', #14092 ) ;
#33175=VERTEX_POINT ( 'NONE', #34336 ) ;
#33207=CARTESIAN_POINT ( 'NONE',  ( 9.132817075745611705E-16, 9.026346327358515609, 0.000000000000000000 ) ) ;
#33222=CARTESIAN_POINT ( 'NONE',  ( 0.000000000000000000, 0.000000000000000000, 0.000000000000000000 ) ) ;
#33233=FACE_OUTER_BOUND ( 'NONE', #28349, .T. ) ;
#33479=FACE_OUTER_BOUND ( 'NONE', #13722, .T. ) ;
#33612=DIRECTION ( 'NONE',  ( -1.000000000000000000, 1.011795553208986254E-16, 0.000000000000000000 ) ) ;
#33627=DIRECTION ( 'NONE',  ( 1.000000000000000000, -1.044409991968847179E-16, 0.000000000000000000 ) ) ;
#33711=DIRECTION ( 'NONE',  ( 1.011795553208986377E-16, 1.000000000000000000, -0.000000000000000000 ) ) ;
#33761=VERTEX_POINT ( 'NONE', #2033 ) ;
#33796=ORIENTED_EDGE ( 'NONE', *, *, #15991, .F. ) ;
#33834=FACE_OUTER_BOUND ( 'NONE', #22608, .T. ) ;
#33916=DIRECTION ( 'NONE',  ( -1.011795553208986377E-16, -1.000000000000000000, 0.000000000000000000 ) ) ;
#33930=AXIS2_PLACEMENT_3D ( 'NONE', #5443, #6277, #25015 ) ;
#34285=AXIS2_PLACEMENT_3D ( 'NONE', #35642, #9235, #2646 ) ;
#34287=ORIENTED_EDGE ( 'NONE', *, *, #20181, .T. ) ;
#34336=CARTESIAN_POINT ( 'NONE',  ( 12.69999999999999929, 14.60500000000000043, 0.000000000000000000 ) ) ;
#34367=EDGE_LOOP ( 'NONE', ( #9017, #14395, #25528, #35537 ) ) ;
#34449=DIRECTION ( 'NONE',  ( 1.000000000000000000, -1.288607544181256449E-16, 0.000000000000000000 ) ) ;
#34455=EDGE_CURVE ( 'NONE', #588, #41686, #36501, .T. ) ;
#34463=ORIENTED_EDGE ( 'NONE', *, *, #36513, .T. ) ;
#34506=AXIS2_PLACEMENT_3D ( 'NONE', #32299, #3129, #35088 ) ;
#34517=ADVANCED_FACE ( 'NONE', ( #39276 ), #30101, .T. ) ;
#34615=LINE ( 'NONE', #38445, #40738 ) ;
#34725=AXIS2_PLACEMENT_3D ( 'NONE', #10074, #7111, #20069 ) ;
#34813=AXIS2_PLACEMENT_3D ( 'NONE', #24441, #5724, #37445 ) ;
#34929=EDGE_CURVE ( 'NONE', #588, #33761, #26329, .T. ) ;
#34939=EDGE_CURVE ( 'NONE', #28134, #23250, #22194, .T. ) ;
#34950=SURFACE_STYLE_FILL_AREA ( #18517 ) ;
#34977=CARTESIAN_POINT ( 'NONE',  ( 9.132817075745611705E-16, 9.026346327358515609, 0.000000000000000000 ) ) ;
#35065=CARTESIAN_POINT ( 'NONE',  ( 16.60960244842765476, 9.026346327358513832, 0.000000000000000000 ) ) ;
#35088=DIRECTION ( 'NONE',  ( -1.000000000000000000, 1.288607544181256449E-16, 0.000000000000000000 ) ) ;
#35198=EDGE_CURVE ( 'NONE', #41686, #33162, #28323, .T. ) ;
#35291=DIRECTION ( 'NONE',  ( -1.011795553208986377E-16, -1.000000000000000000, 0.000000000000000000 ) ) ;
#35370=ORIENTED_EDGE ( 'NONE', *, *, #29256, .F. ) ;
#35414=ORIENTED_EDGE ( 'NONE', *, *, #34455, .T. ) ;
#35495=APPLICATION_CONTEXT ( 'automotive_design' ) ;
#35537=ORIENTED_EDGE ( 'NONE', *, *, #14938, .F. ) ;
#35570=AXIS2_PLACEMENT_3D ( 'NONE', #26178, #23758, #30167 ) ;
#35576=DIRECTION ( 'NONE',  ( 1.011795553208986377E-16, 1.000000000000000000, -0.000000000000000000 ) ) ;
#35604=COLOUR_RGB ( '', 0.31764706, 0.68627451, 0.89019608) ;
#35642=CARTESIAN_POINT ( 'NONE',  ( 9.132817075745611705E-16, 9.026346327358515609, 0.000000000000000000 ) ) ;
#35845=TOROIDAL_SURFACE ( 'NONE', #3898, 16.60960244842765832, 1.396999999999998909 ) ;
#35896=ORIENTED_EDGE ( 'NONE', *, *, #6536, .T. ) ;
#35990=( NAMED_UNIT ( * ) PLANE_ANGLE_UNIT ( ) SI_UNIT ( $, .RADIAN. ) );
#36442=CARTESIAN_POINT ( 'NONE',  ( 1.477727405461724555E-15, 14.60500000000000220, 0.000000000000000000 ) ) ;
#36461=CARTESIAN_POINT ( 'NONE',  ( 1.167505706004672243E-15, 11.53894877578617084, 0.000000000000000000 ) ) ;
#36501=LINE ( 'NONE', #3930, #38545 ) ;
#36513=EDGE_CURVE ( 'NONE', #28134, #10936, #8741, .T. ) ;
#36601=DIRECTION ( 'NONE',  ( 1.011795553208986377E-16, 1.000000000000000000, -0.000000000000000000 ) ) ;
#36916=CIRCLE ( 'NONE', #35570, 15.21260244842765452 ) ;
#37049=DIRECTION ( 'NONE',  ( -1.224646799147353207E-16, 1.239092185628910643E-32, 1.000000000000000000 ) ) ;
#37445=DIRECTION ( 'NONE',  ( -1.000000000000000000, 1.365923996832131856E-16, 0.000000000000000000 ) ) ;
#37495=( LENGTH_UNIT ( ) NAMED_UNIT ( * ) SI_UNIT ( .MILLI., .METRE. ) );
#37662=PLANE ( 'NONE',  #23219 ) ;
#37731=( LENGTH_UNIT ( ) NAMED_UNIT ( * ) SI_UNIT ( .MILLI., .METRE. ) );
#38023=ORIENTED_EDGE ( 'NONE', *, *, #13028, .F. ) ;
#38160=FILL_AREA_STYLE ('',( #24728 ) ) ;
#38209=ORIENTED_EDGE ( 'NONE', *, *, #20410, .T. ) ;
#38309=( GEOMETRIC_REPRESENTATION_CONTEXT ( 3 ) GLOBAL_UNCERTAINTY_ASSIGNED_CONTEXT ( ( #3137 ) ) GLOBAL_UNIT_ASSIGNED_CONTEXT ( ( #37495, #35990, #6389 ) ) REPRESENTATION_CONTEXT ( 'NONE', 'WORKASPACE' ) );
#38322=AXIS2_PLACEMENT_3D ( 'NONE', #33207, #17829, #33627 ) ;
#38350=SURFACE_SIDE_STYLE ('',( #34950 ) ) ;
#38422=VERTEX_POINT ( 'NONE', #21022 ) ;
#38445=CARTESIAN_POINT ( 'NONE',  ( -16.60960244842765832, 17.14499999999999957, 0.000000000000000000 ) ) ;
#38487=DIRECTION ( 'NONE',  ( 1.000000000000000000, -1.044409991968847179E-16, 0.000000000000000000 ) ) ;
#38497=UNCERTAINTY_MEASURE_WITH_UNIT (LENGTH_MEASURE( 1.000000000000000082E-05 ), #8767, 'distance_accuracy_value', 'NONE');
#38545=VECTOR ( 'NONE', #941, 1000.000000000000000 ) ;
#38843=ORIENTED_EDGE ( 'NONE', *, *, #5865, .F. ) ;
#38857=DIRECTION ( 'NONE',  ( 1.011795553208986377E-16, 1.000000000000000000, -0.000000000000000000 ) ) ;
#38886=ORIENTED_EDGE ( 'NONE', *, *, #34929, .T. ) ;
#38918=EDGE_CURVE ( 'NONE', #9144, #31688, #26897, .T. ) ;
#38951=EDGE_CURVE ( 'NONE', #19534, #24265, #39128, .T. ) ;
#39006=CIRCLE ( 'NONE', #39687, 16.60960244842765832 ) ;
#39033=ORIENTED_EDGE ( 'NONE', *, *, #29256, .T. ) ;
#39128=CIRCLE ( 'NONE', #27570, 18.00660244842765323 ) ;
#39208=EDGE_CURVE ( 'NONE', #22322, #19534, #22792, .T. ) ;
#39268=FACE_OUTER_BOUND ( 'NONE', #29029, .T. ) ;
#39276=FACE_OUTER_BOUND ( 'NONE', #14189, .T. ) ;
#39414=ORIENTED_EDGE ( 'NONE', *, *, #23212, .F. ) ;
#39468=DIRECTION ( 'NONE',  ( 1.000000000000000000, 0.000000000000000000, 0.000000000000000000 ) ) ;
#39589=CIRCLE ( 'NONE', #34813, 12.69999999999999751 ) ;
#39599=CARTESIAN_POINT ( 'NONE',  ( 1.400628584307200167E-15, 13.84300000000000352, 0.000000000000000000 ) ) ;
#39687=AXIS2_PLACEMENT_3D ( 'NONE', #33222, #5096, #1689 ) ;
#40070=PRODUCT_DEFINITION_FORMATION_WITH_SPECIFIED_SOURCE ( 'ANY', '', #1125, .NOT_KNOWN. ) ;
#40151=CARTESIAN_POINT ( 'NONE',  ( -13.46199999999999442, 12.17394877578617240, 1.841354584184931751E-15 ) ) ;
#40216=ORIENTED_EDGE ( 'NONE', *, *, #38951, .T. ) ;
#40222=DIRECTION ( 'NONE',  ( 1.011795553208986377E-16, 1.000000000000000000, -0.000000000000000000 ) ) ;
#40227=CARTESIAN_POINT ( 'NONE',  ( 13.46199999999999797, 13.84300000000000175, 0.000000000000000000 ) ) ;
#40282=ADVANCED_FACE ( 'NONE', ( #6301 ), #20211, .F. ) ;
#40324=FACE_OUTER_BOUND ( 'NONE', #10279, .T. ) ;
#40431=ORIENTED_EDGE ( 'NONE', *, *, #13028, .T. ) ;
#40597=ORIENTED_EDGE ( 'NONE', *, *, #198, .T. ) ;
#40634=CARTESIAN_POINT ( 'NONE',  ( 1.400628584307200167E-15, 13.84300000000000352, 0.000000000000000000 ) ) ;
#40738=VECTOR ( 'NONE', #38857, 1000.000000000000000 ) ;
#40785=VERTEX_POINT ( 'NONE', #29503 ) ;
#40991=VECTOR ( 'NONE', #22594, 1000.000000000000000 ) ;
#41124=FILL_AREA_STYLE_COLOUR ( '', #35604 ) ;
#41142=ORIENTED_EDGE ( 'NONE', *, *, #27436, .T. ) ;
#41493=AXIS2_PLACEMENT_3D ( 'NONE', #24826, #31647, #15450 ) ;
#41686=VERTEX_POINT ( 'NONE', #6769 ) ;
#41846=ORIENTED_EDGE ( 'NONE', *, *, #29867, .T. ) ;
#41934=EDGE_LOOP ( 'NONE', ( #25255, #32563, #11949, #10741 ) ) ;
#41999=ORIENTED_EDGE ( 'NONE', *, *, #10985, .T. ) ;
ENDSEC;
END-ISO-10303-21;
